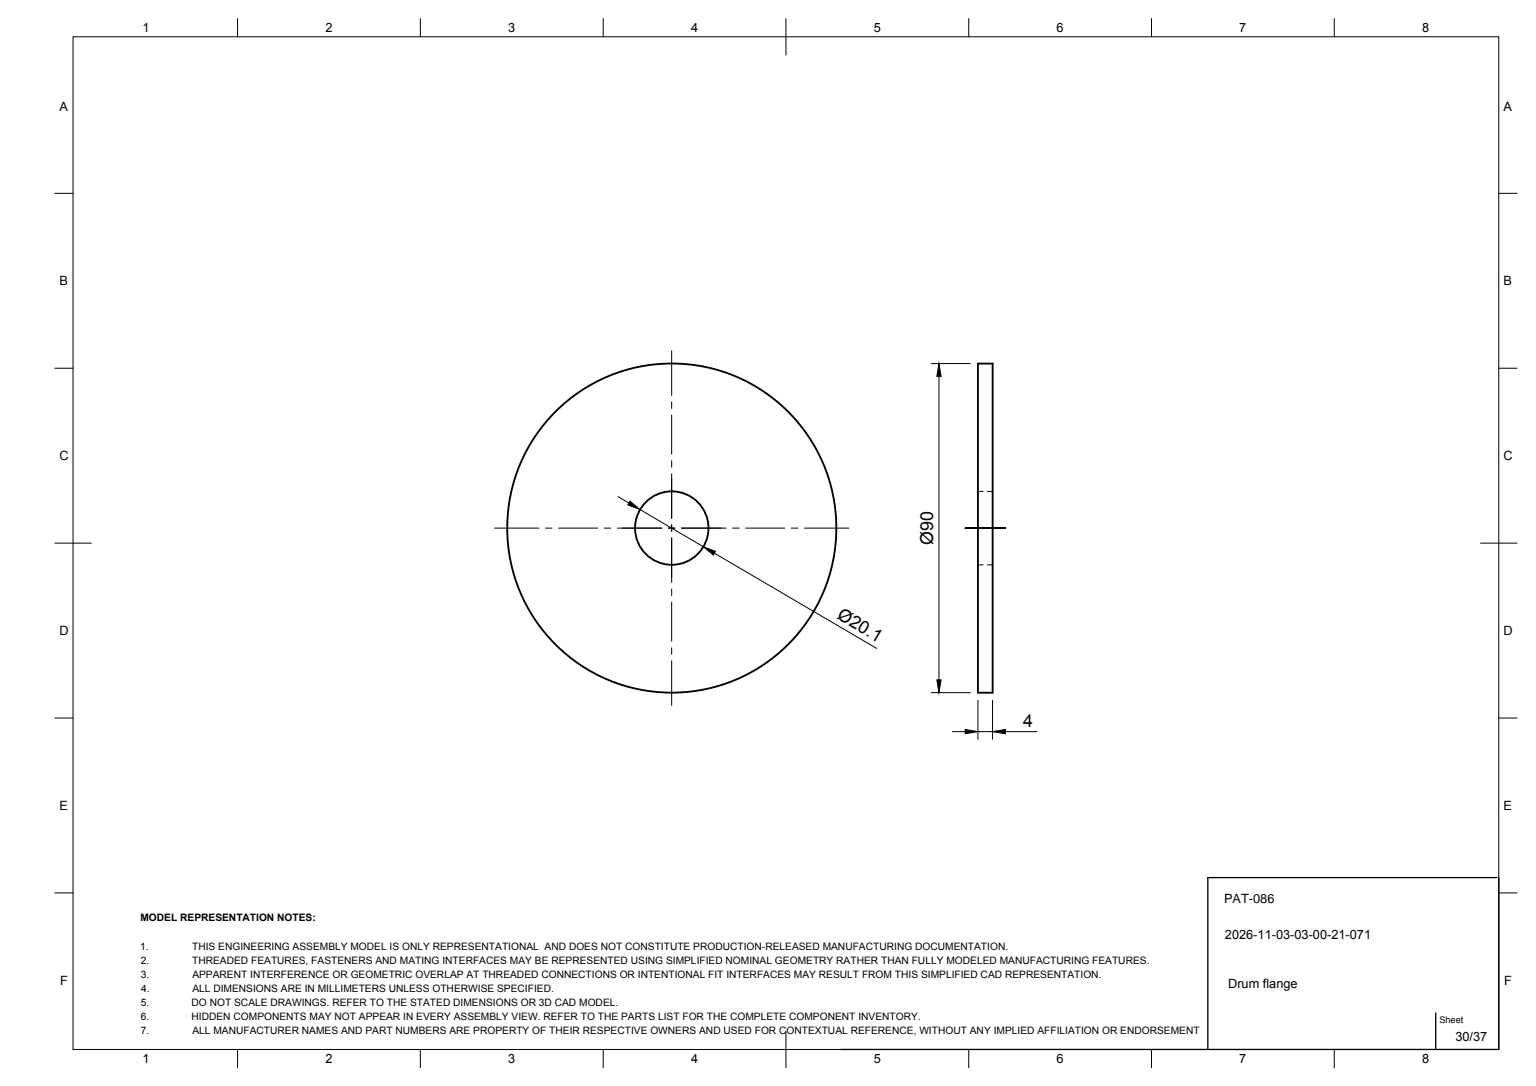
ISO-10303-21;
HEADER;
/* Generated by software containing ST-Developer
 * from STEP Tools, Inc. (www.steptools.com) 
 */

FILE_DESCRIPTION(
/* description */ ('Ratchet and pawl hand winch drum'),
/* implementation_level */ '2;1');

FILE_NAME(
/* name */ 'Drum flange.step',
/* time_stamp */ '2026-10-27T12:42:58-07:00',
/* author */ (''),
/* organization */ (''),
/* preprocessor_version */ 'ST-DEVELOPER v20.2',
/* originating_system */ 'Autodesk Translation Framework v15.17.0.0',
/* authorisation */ '');

FILE_SCHEMA (('AUTOMOTIVE_DESIGN { 1 0 10303 214 3 1 1 }'));
ENDSEC;

DATA;
#10=MECHANICAL_DESIGN_GEOMETRIC_PRESENTATION_REPRESENTATION('',(#414),#11801);
#345=SHAPE_REPRESENTATION_RELATIONSHIP('SRR','None',#11973,#379);
#379=ADVANCED_BREP_SHAPE_REPRESENTATION('',(#447),#11790);
#414=STYLED_ITEM('',(#12199),#447);
#447=MANIFOLD_SOLID_BREP('Body1',#6293);
#574=FACE_BOUND('',#1541,.T.);
#575=FACE_BOUND('',#1543,.T.);
#738=PLANE('',#7102);
#739=PLANE('',#7103);
#1064=FACE_OUTER_BOUND('',#1538,.T.);
#1065=FACE_OUTER_BOUND('',#1539,.T.);
#1066=FACE_OUTER_BOUND('',#1540,.T.);
#1067=FACE_OUTER_BOUND('',#1542,.T.);
#1538=EDGE_LOOP('',(#5183,#5184,#5185,#5186));
#1539=EDGE_LOOP('',(#5187,#5188,#5189,#5190));
#1540=EDGE_LOOP('',(#5191));
#1541=EDGE_LOOP('',(#5192));
#1542=EDGE_LOOP('',(#5193));
#1543=EDGE_LOOP('',(#5194));
#1971=LINE('',#10800,#2482);
#1972=LINE('',#10806,#2483);
#2482=VECTOR('',#8470,1.005);
#2483=VECTOR('',#8477,4.5);
#2881=CIRCLE('',#7097,1.005);
#2882=CIRCLE('',#7098,1.005);
#2883=CIRCLE('',#7100,4.5);
#2884=CIRCLE('',#7101,4.5);
#3260=VERTEX_POINT('',#10797);
#3261=VERTEX_POINT('',#10799);
#3262=VERTEX_POINT('',#10803);
#3263=VERTEX_POINT('',#10805);
#3935=EDGE_CURVE('',#3260,#3260,#2881,.T.);
#3936=EDGE_CURVE('',#3260,#3261,#1971,.T.);
#3937=EDGE_CURVE('',#3261,#3261,#2882,.T.);
#3938=EDGE_CURVE('',#3262,#3262,#2883,.T.);
#3939=EDGE_CURVE('',#3262,#3263,#1972,.T.);
#3940=EDGE_CURVE('',#3263,#3263,#2884,.T.);
#5183=ORIENTED_EDGE('',*,*,#3935,.F.);
#5184=ORIENTED_EDGE('',*,*,#3936,.T.);
#5185=ORIENTED_EDGE('',*,*,#3937,.T.);
#5186=ORIENTED_EDGE('',*,*,#3936,.F.);
#5187=ORIENTED_EDGE('',*,*,#3938,.F.);
#5188=ORIENTED_EDGE('',*,*,#3939,.T.);
#5189=ORIENTED_EDGE('',*,*,#3940,.T.);
#5190=ORIENTED_EDGE('',*,*,#3939,.F.);
#5191=ORIENTED_EDGE('',*,*,#3938,.T.);
#5192=ORIENTED_EDGE('',*,*,#3935,.T.);
#5193=ORIENTED_EDGE('',*,*,#3940,.F.);
#5194=ORIENTED_EDGE('',*,*,#3937,.F.);
#5886=CYLINDRICAL_SURFACE('',#7096,1.005);
#5887=CYLINDRICAL_SURFACE('',#7099,4.5);
#6134=ADVANCED_FACE('',(#1064),#5886,.F.);
#6135=ADVANCED_FACE('',(#1065),#5887,.T.);
#6136=ADVANCED_FACE('',(#1066,#574),#738,.T.);
#6137=ADVANCED_FACE('',(#1067,#575),#739,.F.);
#6293=CLOSED_SHELL('',(#6134,#6135,#6136,#6137));
#7095=AXIS2_PLACEMENT_3D('',#10795,#8464,#8465);
#7096=AXIS2_PLACEMENT_3D('',#10796,#8466,#8467);
#7097=AXIS2_PLACEMENT_3D('',#10798,#8468,#8469);
#7098=AXIS2_PLACEMENT_3D('',#10801,#8471,#8472);
#7099=AXIS2_PLACEMENT_3D('',#10802,#8473,#8474);
#7100=AXIS2_PLACEMENT_3D('',#10804,#8475,#8476);
#7101=AXIS2_PLACEMENT_3D('',#10807,#8478,#8479);
#7102=AXIS2_PLACEMENT_3D('',#10808,#8480,#8481);
#7103=AXIS2_PLACEMENT_3D('',#10809,#8482,#8483);
#8464=DIRECTION('axis',(0.,0.,1.));
#8465=DIRECTION('refdir',(1.,0.,0.));
#8466=DIRECTION('center_axis',(0.,1.,0.));
#8467=DIRECTION('ref_axis',(1.,0.,0.));
#8468=DIRECTION('center_axis',(0.,-1.,0.));
#8469=DIRECTION('ref_axis',(1.,0.,0.));
#8470=DIRECTION('',(0.,-1.,0.));
#8471=DIRECTION('center_axis',(0.,-1.,0.));
#8472=DIRECTION('ref_axis',(1.,0.,0.));
#8473=DIRECTION('center_axis',(0.,1.,0.));
#8474=DIRECTION('ref_axis',(1.,0.,0.));
#8475=DIRECTION('center_axis',(0.,1.,0.));
#8476=DIRECTION('ref_axis',(1.,0.,0.));
#8477=DIRECTION('',(0.,-1.,0.));
#8478=DIRECTION('center_axis',(0.,1.,0.));
#8479=DIRECTION('ref_axis',(1.,0.,0.));
#8480=DIRECTION('center_axis',(0.,1.,0.));
#8481=DIRECTION('ref_axis',(1.,0.,0.));
#8482=DIRECTION('center_axis',(0.,1.,0.));
#8483=DIRECTION('ref_axis',(1.,0.,0.));
#10795=CARTESIAN_POINT('',(0.,0.,0.));
#10796=CARTESIAN_POINT('Origin',(0.,2.6,6.53));
#10797=CARTESIAN_POINT('',(-1.005,3.,6.53));
#10798=CARTESIAN_POINT('Origin',(0.,3.,6.53));
#10799=CARTESIAN_POINT('',(-1.005,2.6,6.53));
#10800=CARTESIAN_POINT('',(-1.005,2.6,6.53));
#10801=CARTESIAN_POINT('Origin',(0.,2.6,6.53));
#10802=CARTESIAN_POINT('Origin',(0.,2.6,6.53));
#10803=CARTESIAN_POINT('',(-4.5,3.,6.53));
#10804=CARTESIAN_POINT('Origin',(0.,3.,6.53));
#10805=CARTESIAN_POINT('',(-4.5,2.6,6.53));
#10806=CARTESIAN_POINT('',(-4.5,2.6,6.53));
#10807=CARTESIAN_POINT('Origin',(0.,2.6,6.53));
#10808=CARTESIAN_POINT('Origin',(0.,3.,6.53));
#10809=CARTESIAN_POINT('Origin',(0.,2.6,6.53));
#11750=UNCERTAINTY_MEASURE_WITH_UNIT(LENGTH_MEASURE(0.001),#11802,
'DISTANCE_ACCURACY_VALUE',
'Maximum model space distance between geometric entities at asserted c
onnectivities');
#11761=UNCERTAINTY_MEASURE_WITH_UNIT(LENGTH_MEASURE(0.001),#11802,
'DISTANCE_ACCURACY_VALUE',
'Maximum model space distance between geometric entities at asserted c
onnectivities');
#11790=(
GEOMETRIC_REPRESENTATION_CONTEXT(3)
GLOBAL_UNCERTAINTY_ASSIGNED_CONTEXT((#11750))
GLOBAL_UNIT_ASSIGNED_CONTEXT((#11802,#11804,#11805))
REPRESENTATION_CONTEXT('','3D')
);
#11801=(
GEOMETRIC_REPRESENTATION_CONTEXT(3)
GLOBAL_UNCERTAINTY_ASSIGNED_CONTEXT((#11761))
GLOBAL_UNIT_ASSIGNED_CONTEXT((#11802,#11804,#11805))
REPRESENTATION_CONTEXT('','3D')
);
#11802=(
LENGTH_UNIT()
NAMED_UNIT(*)
SI_UNIT(.CENTI.,.METRE.)
);
#11804=(
NAMED_UNIT(*)
PLANE_ANGLE_UNIT()
SI_UNIT($,.RADIAN.)
);
#11805=(
NAMED_UNIT(*)
SI_UNIT($,.STERADIAN.)
SOLID_ANGLE_UNIT()
);
#11834=SHAPE_DEFINITION_REPRESENTATION(#11875,#11973);
#11875=PRODUCT_DEFINITION_SHAPE('',$,#12013);
#11973=SHAPE_REPRESENTATION('',(#7095),#11790);
#11984=PRODUCT_DEFINITION_CONTEXT('part definition',#12103,'design');
#12013=PRODUCT_DEFINITION('Drum flange','Drum flange',#12052,#11984);
#12052=PRODUCT_DEFINITION_FORMATION('',$,#12133);
#12103=APPLICATION_CONTEXT(
'Core Data for Automotive Mechanical Design Process');
#12104=PRODUCT_CONTEXT('part definition',#12103,'mechanical');
#12133=PRODUCT('Drum flange','Drum flange','Drum flange',(#12104));
#12193=COLOUR_RGB('Light Blue',0.38,0.62,0.78);
#12194=FILL_AREA_STYLE_COLOUR('',#12193);
#12195=FILL_AREA_STYLE('',(#12194));
#12196=SURFACE_STYLE_FILL_AREA(#12195);
#12197=SURFACE_SIDE_STYLE('',(#12196));
#12198=SURFACE_STYLE_USAGE(.BOTH.,#12197);
#12199=PRESENTATION_STYLE_ASSIGNMENT((#12198));
ENDSEC;
END-ISO-10303-21;
